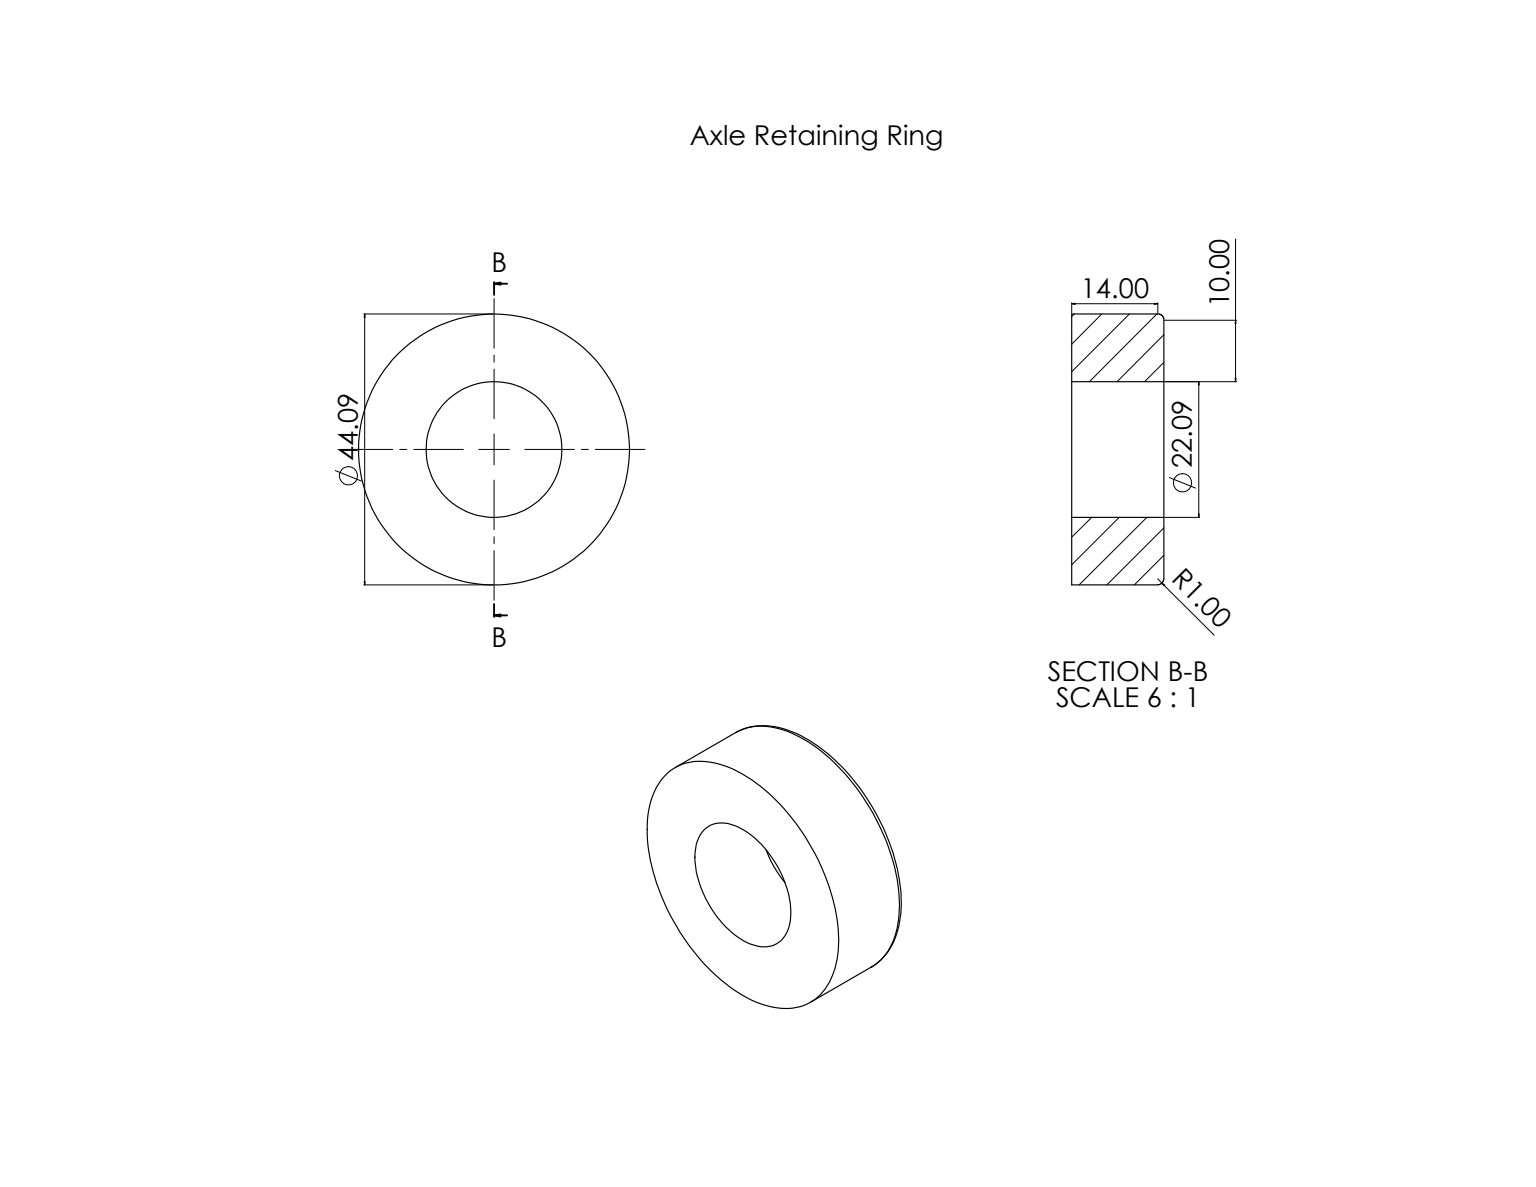
ISO-10303-21;
HEADER;
FILE_DESCRIPTION (('STEP AP214'),
    '1' );
FILE_NAME ('Axle Retaining Ring.step',
    '2026-10-21T18:33:49',
    ( '' ),
    ( '' ),
    'SwSTEP 2.0',
    'SolidWorks 2025',
    '' );
FILE_SCHEMA (( 'AUTOMOTIVE_DESIGN' ));
ENDSEC;

DATA;
#55=CIRCLE ( 'NONE', #2439, 22.04359719766050318 ) ;
#64=FACE_OUTER_BOUND ( 'NONE', #11864, .T. ) ;
#89=ORIENTED_EDGE ( 'NONE', *, *, #17144, .T. ) ;
#192=CYLINDRICAL_SURFACE ( 'NONE', #914, 11.04359719766050141 ) ;
#240=DIRECTION ( 'NONE',  ( 1.000000000000000000, 0.000000000000000000, 0.000000000000000000 ) ) ;
#257=MANIFOLD_SOLID_BREP ( 'Fillet4', #11497 ) ;
#347=SHAPE_REPRESENTATION_RELATIONSHIP ( 'NONE' , 'NONE' ,  #8623, #5245 ) ;
#437=ORIENTED_EDGE ( 'NONE', *, *, #1963, .T. ) ;
#454=DIRECTION ( 'NONE',  ( 0.000000000000000000, 0.000000000000000000, -1.000000000000000000 ) ) ;
#484=DIRECTION ( 'NONE',  ( 0.000000000000000000, 0.000000000000000000, -1.000000000000000000 ) ) ;
#549=FACE_OUTER_BOUND ( 'NONE', #11506, .T. ) ;
#746=DIRECTION ( 'NONE',  ( 0.000000000000000000, 0.000000000000000000, -1.000000000000000000 ) ) ;
#889=VERTEX_POINT ( 'NONE', #11533 ) ;
#914=AXIS2_PLACEMENT_3D ( 'NONE', #4475, #8427, #7036 ) ;
#1034=AXIS2_PLACEMENT_3D ( 'NONE', #3289, #4973, #4881 ) ;
#1044=DIRECTION ( 'NONE',  ( -1.000000000000000000, 0.000000000000000000, -0.000000000000000000 ) ) ;
#1046=STYLED_ITEM('',(#18559),#257);
#1223=CIRCLE ( 'NONE', #15253, 1.000000000000000888 ) ;
#1313=AXIS2_PLACEMENT_3D ( 'NONE', #12912, #7285, #17108 ) ;
#1444=EDGE_LOOP ( 'NONE', ( #12591, #14406, #8413, #6180 ) ) ;
#1515=DIRECTION ( 'NONE',  ( 1.000000000000000000, 0.000000000000000000, 0.000000000000000000 ) ) ;
#1526=VERTEX_POINT ( 'NONE', #2815 ) ;
#1551=DIRECTION ( 'NONE',  ( 0.000000000000000000, 0.000000000000000000, -1.000000000000000000 ) ) ;
#1578=DIRECTION ( 'NONE',  ( -1.224646799147353207E-16, 1.000000000000000000, 0.000000000000000000 ) ) ;
#1585=FACE_OUTER_BOUND ( 'NONE', #1876, .T. ) ;
#1605=FACE_OUTER_BOUND ( 'NONE', #1444, .T. ) ;
#1668=( NAMED_UNIT ( * ) PLANE_ANGLE_UNIT ( ) SI_UNIT ( $, .RADIAN. ) );
#1876=EDGE_LOOP ( 'NONE', ( #12983, #14667, #10558, #5358 ) ) ;
#1963=EDGE_CURVE ( 'NONE', #1526, #6914, #14518, .T. ) ;
#1995=EDGE_LOOP ( 'NONE', ( #11913, #4157 ) ) ;
#2070=AXIS2_PLACEMENT_3D ( 'NONE', #14552, #10073, #15773 ) ;
#2156=EDGE_CURVE ( 'NONE', #6914, #1526, #8158, .T. ) ;
#2191=VERTEX_POINT ( 'NONE', #5122 ) ;
#2398=DIRECTION ( 'NONE',  ( 0.000000000000000000, 0.000000000000000000, -1.000000000000000000 ) ) ;
#2439=AXIS2_PLACEMENT_3D ( 'NONE', #17290, #454, #8698 ) ;
#2806=AXIS2_PLACEMENT_3D ( 'NONE', #15914, #3105, #8818 ) ;
#2815=CARTESIAN_POINT ( 'NONE',  ( -46.03642545851250389, 84.22855780814606419, -47.50000000000000000 ) ) ;
#2834=CARTESIAN_POINT ( 'NONE',  ( -79.12361985383350316, 84.22855780814606419, -124.8487082408420861 ) ) ;
#2847=CARTESIAN_POINT ( 'NONE',  ( -57.08002265617300708, 84.22855780814606419, -61.50000000000000000 ) ) ;
#3105=DIRECTION ( 'NONE',  ( -0.000000000000000000, -0.000000000000000000, 1.000000000000000000 ) ) ;
#3289=CARTESIAN_POINT ( 'NONE',  ( -57.08002265617300708, 84.22855780814606419, -47.50000000000000000 ) ) ;
#3354=DIRECTION ( 'NONE',  ( 0.000000000000000000, 0.000000000000000000, -1.000000000000000000 ) ) ;
#3361=CARTESIAN_POINT ( 'NONE',  ( -68.12361985383350316, 84.22855780814606419, -124.8487082408420861 ) ) ;
#3368=DIRECTION ( 'NONE',  ( -1.000000000000000000, 0.000000000000000000, 0.000000000000000000 ) ) ;
#3372=AXIS2_PLACEMENT_3D ( 'NONE', #8660, #1551, #7259 ) ;
#3376=EDGE_CURVE ( 'NONE', #9602, #3839, #4404, .T. ) ;
#3486=ORIENTED_EDGE ( 'NONE', *, *, #18487, .F. ) ;
#3634=DIRECTION ( 'NONE',  ( -1.000000000000000000, 0.000000000000000000, 0.000000000000000000 ) ) ;
#3662=TOROIDAL_SURFACE ( 'NONE', #17400, 21.04359719766050674, 1.000000000000000000 ) ;
#3703=APPLICATION_CONTEXT ( 'automotive_design' ) ;
#3801=EDGE_CURVE ( 'NONE', #16706, #10794, #15822, .T. ) ;
#3839=VERTEX_POINT ( 'NONE', #7263 ) ;
#3840=PRODUCT_DEFINITION_CONTEXT ( 'detailed design', #3703, 'design' ) ;
#4157=ORIENTED_EDGE ( 'NONE', *, *, #3801, .T. ) ;
#4322=CYLINDRICAL_SURFACE ( 'NONE', #11999, 11.04359719766050141 ) ;
#4404=LINE ( 'NONE', #2834, #14606 ) ;
#4475=CARTESIAN_POINT ( 'NONE',  ( -57.08002265617300708, 84.22855780814606419, -124.8487082408420861 ) ) ;
#4610=CARTESIAN_POINT ( 'NONE',  ( -36.03642545851250389, 84.22855780814606419, -62.50000000000000000 ) ) ;
#4741=ADVANCED_FACE ( 'NONE', ( #5238, #6539 ), #16548, .T. ) ;
#4748=CARTESIAN_POINT ( 'NONE',  ( -57.08002265617300708, 84.22855780814606419, -47.50000000000000000 ) ) ;
#4881=DIRECTION ( 'NONE',  ( -1.000000000000000000, 0.000000000000000000, 0.000000000000000000 ) ) ;
#4901=ADVANCED_FACE ( 'NONE', ( #1585 ), #192, .F. ) ;
#4973=DIRECTION ( 'NONE',  ( 0.000000000000000000, 0.000000000000000000, -1.000000000000000000 ) ) ;
#5109=CARTESIAN_POINT ( 'NONE',  ( -78.12361985383350316, 84.22855780814606419, -61.50000000000000000 ) ) ;
#5122=CARTESIAN_POINT ( 'NONE',  ( -35.03642545851250389, 84.22855780814606419, -47.50000000000000000 ) ) ;
#5238=FACE_OUTER_BOUND ( 'NONE', #1995, .T. ) ;
#5245=ADVANCED_BREP_SHAPE_REPRESENTATION ( '', ( #257, #16217 ), #8171 ) ;
#5358=ORIENTED_EDGE ( 'NONE', *, *, #6020, .F. ) ;
#5466=CARTESIAN_POINT ( 'NONE',  ( -57.08002265617300708, 84.22855780814606419, -61.50000000000000000 ) ) ;
#5480=FACE_OUTER_BOUND ( 'NONE', #11849, .T. ) ;
#5519=AXIS2_PLACEMENT_3D ( 'NONE', #11491, #10346, #240 ) ;
#5637=ADVANCED_FACE ( 'NONE', ( #8637 ), #6191, .T. ) ;
#5675=EDGE_CURVE ( 'NONE', #3839, #2191, #17875, .T. ) ;
#5714=DIRECTION ( 'NONE',  ( -0.000000000000000000, -0.000000000000000000, 1.000000000000000000 ) ) ;
#5762=CYLINDRICAL_SURFACE ( 'NONE', #5519, 22.04359719766050318 ) ;
#5781=CARTESIAN_POINT ( 'NONE',  ( 0.000000000000000000, 0.000000000000000000, 0.000000000000000000 ) ) ;
#6020=EDGE_CURVE ( 'NONE', #9668, #1526, #13101, .T. ) ;
#6037=DIRECTION ( 'NONE',  ( 0.000000000000000000, 0.000000000000000000, 1.000000000000000000 ) ) ;
#6080=ORIENTED_EDGE ( 'NONE', *, *, #5675, .F. ) ;
#6180=ORIENTED_EDGE ( 'NONE', *, *, #2156, .F. ) ;
#6191=TOROIDAL_SURFACE ( 'NONE', #8622, 21.04359719766050674, 1.000000000000000000 ) ;
#6239=FACE_BOUND ( 'NONE', #11509, .T. ) ;
#6318=AXIS2_PLACEMENT_3D ( 'NONE', #5109, #15216, #2398 ) ;
#6347=VECTOR ( 'NONE', #13665, 1000.000000000000000 ) ;
#6352=CARTESIAN_POINT ( 'NONE',  ( -57.08002265617300708, 84.22855780814606419, -47.50000000000000000 ) ) ;
#6539=FACE_BOUND ( 'NONE', #11372, .T. ) ;
#6635=CARTESIAN_POINT ( 'NONE',  ( -46.03642545851250389, 84.22855780814606419, -62.50000000000000000 ) ) ;
#6740=CARTESIAN_POINT ( 'NONE',  ( -57.08002265617300708, 84.22855780814606419, -62.50000000000000000 ) ) ;
#6791=DIRECTION ( 'NONE',  ( -1.000000000000000000, 0.000000000000000000, -0.000000000000000000 ) ) ;
#6908=CIRCLE ( 'NONE', #12272, 22.04359719766050318 ) ;
#6914=VERTEX_POINT ( 'NONE', #16473 ) ;
#6923=CARTESIAN_POINT ( 'NONE',  ( -57.08002265617300708, 84.22855780814606419, -62.50000000000000000 ) ) ;
#7006=ORIENTED_EDGE ( 'NONE', *, *, #2156, .T. ) ;
#7012=DIRECTION ( 'NONE',  ( -0.000000000000000000, -0.000000000000000000, 1.000000000000000000 ) ) ;
#7036=DIRECTION ( 'NONE',  ( 1.000000000000000000, 0.000000000000000000, 0.000000000000000000 ) ) ;
#7099=LINE ( 'NONE', #18230, #12890 ) ;
#7259=DIRECTION ( 'NONE',  ( -1.000000000000000000, 0.000000000000000000, 0.000000000000000000 ) ) ;
#7263=CARTESIAN_POINT ( 'NONE',  ( -79.12361985383350316, 84.22855780814606419, -47.50000000000000000 ) ) ;
#7285=DIRECTION ( 'NONE',  ( 0.000000000000000000, 0.000000000000000000, -1.000000000000000000 ) ) ;
#7460=CARTESIAN_POINT ( 'NONE',  ( -57.08002265617300708, 84.22855780814606419, -61.50000000000000000 ) ) ;
#7481=PRODUCT_DEFINITION ( 'UNKNOWN', '', #9987, #3840 ) ;
#7550=( NAMED_UNIT ( * ) SI_UNIT ( $, .STERADIAN. ) SOLID_ANGLE_UNIT ( ) );
#7708=ORIENTED_EDGE ( 'NONE', *, *, #14542, .T. ) ;
#7914=CIRCLE ( 'NONE', #18390, 21.04359719766050318 ) ;
#7960=ORIENTED_EDGE ( 'NONE', *, *, #17144, .F. ) ;
#8036=DIRECTION ( 'NONE',  ( 0.000000000000000000, 0.000000000000000000, -1.000000000000000000 ) ) ;
#8158=CIRCLE ( 'NONE', #9073, 11.04359719766049430 ) ;
#8171=( GEOMETRIC_REPRESENTATION_CONTEXT ( 3 ) GLOBAL_UNCERTAINTY_ASSIGNED_CONTEXT ( ( #18256 ) ) GLOBAL_UNIT_ASSIGNED_CONTEXT ( ( #11672, #1668, #7550 ) ) REPRESENTATION_CONTEXT ( 'NONE', 'WORKASPACE' ) );
#8413=ORIENTED_EDGE ( 'NONE', *, *, #6020, .T. ) ;
#8425=CARTESIAN_POINT ( 'NONE',  ( -79.12361985383350316, 84.22855780814606419, -61.50000000000000000 ) ) ;
#8427=DIRECTION ( 'NONE',  ( -0.000000000000000000, -0.000000000000000000, 1.000000000000000000 ) ) ;
#8622=AXIS2_PLACEMENT_3D ( 'NONE', #2847, #15920, #17142 ) ;
#8623=SHAPE_REPRESENTATION ( 'Axle Retaining Ring', ( #16217 ), #8171 ) ;
#8630=ORIENTED_EDGE ( 'NONE', *, *, #12433, .F. ) ;
#8637=FACE_OUTER_BOUND ( 'NONE', #14875, .T. ) ;
#8660=CARTESIAN_POINT ( 'NONE',  ( -57.08002265617300708, 84.22855780814606419, -62.50000000000000000 ) ) ;
#8698=DIRECTION ( 'NONE',  ( -1.000000000000000000, 0.000000000000000000, 0.000000000000000000 ) ) ;
#8803=MECHANICAL_DESIGN_GEOMETRIC_PRESENTATION_REPRESENTATION('',(#1046),#17447);
#8818=DIRECTION ( 'NONE',  ( -1.000000000000000000, 0.000000000000000000, 0.000000000000000000 ) ) ;
#8961=DIRECTION ( 'NONE',  ( 1.000000000000000000, 0.000000000000000000, 0.000000000000000000 ) ) ;
#9073=AXIS2_PLACEMENT_3D ( 'NONE', #13654, #746, #17658 ) ;
#9365=ADVANCED_FACE ( 'NONE', ( #1605 ), #4322, .F. ) ;
#9441=APPLICATION_CONTEXT ( 'automotive_design' ) ;
#9448=DIRECTION ( 'NONE',  ( 0.000000000000000000, 0.000000000000000000, -1.000000000000000000 ) ) ;
#9602=VERTEX_POINT ( 'NONE', #8425 ) ;
#9668=VERTEX_POINT ( 'NONE', #6635 ) ;
#9956=( LENGTH_UNIT ( ) NAMED_UNIT ( * ) SI_UNIT ( .MILLI., .METRE. ) );
#9987=PRODUCT_DEFINITION_FORMATION_WITH_SPECIFIED_SOURCE ( 'ANY', '', #17885, .NOT_KNOWN. ) ;
#10046=ORIENTED_EDGE ( 'NONE', *, *, #17180, .T. ) ;
#10073=DIRECTION ( 'NONE',  ( 0.000000000000000000, 0.000000000000000000, -1.000000000000000000 ) ) ;
#10084=ADVANCED_FACE ( 'NONE', ( #18196 ), #3662, .T. ) ;
#10346=DIRECTION ( 'NONE',  ( -0.000000000000000000, -0.000000000000000000, 1.000000000000000000 ) ) ;
#10467=AXIS2_PLACEMENT_3D ( 'NONE', #6740, #8036, #1044 ) ;
#10558=ORIENTED_EDGE ( 'NONE', *, *, #1963, .F. ) ;
#10630=EDGE_CURVE ( 'NONE', #9602, #11331, #14443, .T. ) ;
#10651=EDGE_CURVE ( 'NONE', #889, #6914, #15055, .T. ) ;
#10728=ORIENTED_EDGE ( 'NONE', *, *, #3376, .F. ) ;
#10794=VERTEX_POINT ( 'NONE', #15015 ) ;
#11011=ADVANCED_FACE ( 'NONE', ( #5480 ), #11207, .T. ) ;
#11114=EDGE_CURVE ( 'NONE', #9668, #889, #16838, .T. ) ;
#11207=CYLINDRICAL_SURFACE ( 'NONE', #18036, 22.04359719766050318 ) ;
#11323=ORIENTED_EDGE ( 'NONE', *, *, #15890, .T. ) ;
#11331=VERTEX_POINT ( 'NONE', #11592 ) ;
#11372=EDGE_LOOP ( 'NONE', ( #14308, #3486 ) ) ;
#11428=DIRECTION ( 'NONE',  ( -0.000000000000000000, -0.000000000000000000, 1.000000000000000000 ) ) ;
#11491=CARTESIAN_POINT ( 'NONE',  ( -57.08002265617300708, 84.22855780814606419, -124.8487082408420861 ) ) ;
#11497=CLOSED_SHELL ( 'NONE', ( #5637, #4901, #11011, #11787, #12967, #9365, #4741, #10084 ) ) ;
#11506=EDGE_LOOP ( 'NONE', ( #7960, #6080 ) ) ;
#11509=EDGE_LOOP ( 'NONE', ( #437, #7006 ) ) ;
#11533=CARTESIAN_POINT ( 'NONE',  ( -68.12361985383350316, 84.22855780814606419, -62.50000000000000000 ) ) ;
#11592=CARTESIAN_POINT ( 'NONE',  ( -35.03642545851250389, 84.22855780814606419, -61.50000000000000000 ) ) ;
#11672=( LENGTH_UNIT ( ) NAMED_UNIT ( * ) SI_UNIT ( .MILLI., .METRE. ) );
#11678=CARTESIAN_POINT ( 'NONE',  ( -36.03642545851250389, 84.22855780814606419, -61.50000000000000000 ) ) ;
#11787=ADVANCED_FACE ( 'NONE', ( #64 ), #5762, .T. ) ;
#11849=EDGE_LOOP ( 'NONE', ( #12289, #18252, #13254, #12189 ) ) ;
#11864=EDGE_LOOP ( 'NONE', ( #10728, #13849, #7708, #89 ) ) ;
#11913=ORIENTED_EDGE ( 'NONE', *, *, #12433, .T. ) ;
#11999=AXIS2_PLACEMENT_3D ( 'NONE', #15820, #5714, #1515 ) ;
#12076=ORIENTED_EDGE ( 'NONE', *, *, #15923, .F. ) ;
#12189=ORIENTED_EDGE ( 'NONE', *, *, #14542, .F. ) ;
#12272=AXIS2_PLACEMENT_3D ( 'NONE', #7460, #17283, #14660 ) ;
#12289=ORIENTED_EDGE ( 'NONE', *, *, #15923, .T. ) ;
#12317=CIRCLE ( 'NONE', #6318, 1.000000000000000888 ) ;
#12405=SHAPE_DEFINITION_REPRESENTATION ( #12710, #8623 ) ;
#12433=EDGE_CURVE ( 'NONE', #10794, #16706, #7914, .T. ) ;
#12591=ORIENTED_EDGE ( 'NONE', *, *, #10651, .F. ) ;
#12710=PRODUCT_DEFINITION_SHAPE ( 'NONE', 'NONE',  #7481 ) ;
#12890=VECTOR ( 'NONE', #7012, 1000.000000000000000 ) ;
#12912=CARTESIAN_POINT ( 'NONE',  ( -57.08002265617300708, 84.22855780814606419, -62.50000000000000000 ) ) ;
#12967=ADVANCED_FACE ( 'NONE', ( #549, #6239 ), #17566, .F. ) ;
#12983=ORIENTED_EDGE ( 'NONE', *, *, #11114, .T. ) ;
#13070=DIRECTION ( 'NONE',  ( 1.000000000000000000, 0.000000000000000000, 0.000000000000000000 ) ) ;
#13101=LINE ( 'NONE', #14322, #15796 ) ;
#13254=ORIENTED_EDGE ( 'NONE', *, *, #5675, .T. ) ;
#13299=ORIENTED_EDGE ( 'NONE', *, *, #3801, .F. ) ;
#13391=UNCERTAINTY_MEASURE_WITH_UNIT (LENGTH_MEASURE( 1.000000000000000082E-05 ), #9956, 'distance_accuracy_value', 'NONE');
#13654=CARTESIAN_POINT ( 'NONE',  ( -57.08002265617300708, 84.22855780814606419, -47.50000000000000000 ) ) ;
#13665=DIRECTION ( 'NONE',  ( -0.000000000000000000, -0.000000000000000000, 1.000000000000000000 ) ) ;
#13849=ORIENTED_EDGE ( 'NONE', *, *, #10630, .T. ) ;
#13996=DIRECTION ( 'NONE',  ( -1.000000000000000000, 0.000000000000000000, 0.000000000000000000 ) ) ;
#14308=ORIENTED_EDGE ( 'NONE', *, *, #11114, .F. ) ;
#14322=CARTESIAN_POINT ( 'NONE',  ( -46.03642545851250389, 84.22855780814606419, -124.8487082408420861 ) ) ;
#14406=ORIENTED_EDGE ( 'NONE', *, *, #18487, .T. ) ;
#14443=CIRCLE ( 'NONE', #2806, 22.04359719766050318 ) ;
#14518=CIRCLE ( 'NONE', #1034, 11.04359719766049430 ) ;
#14542=EDGE_CURVE ( 'NONE', #11331, #2191, #7099, .T. ) ;
#14552=CARTESIAN_POINT ( 'NONE',  ( -57.08002265617300708, 84.22855780814606419, -62.50000000000000000 ) ) ;
#14606=VECTOR ( 'NONE', #17301, 1000.000000000000000 ) ;
#14660=DIRECTION ( 'NONE',  ( -1.000000000000000000, 0.000000000000000000, 0.000000000000000000 ) ) ;
#14667=ORIENTED_EDGE ( 'NONE', *, *, #10651, .T. ) ;
#14875=EDGE_LOOP ( 'NONE', ( #12076, #11323, #8630, #16662 ) ) ;
#15015=CARTESIAN_POINT ( 'NONE',  ( -78.12361985383350316, 84.22855780814606419, -62.50000000000000000 ) ) ;
#15055=LINE ( 'NONE', #3361, #6347 ) ;
#15179=PRODUCT_CONTEXT ( 'NONE', #9441, 'mechanical' ) ;
#15216=DIRECTION ( 'NONE',  ( -0.000000000000000000, -1.000000000000000000, -0.000000000000000000 ) ) ;
#15253=AXIS2_PLACEMENT_3D ( 'NONE', #11678, #1578, #17466 ) ;
#15273=ORIENTED_EDGE ( 'NONE', *, *, #15890, .F. ) ;
#15277=( NAMED_UNIT ( * ) PLANE_ANGLE_UNIT ( ) SI_UNIT ( $, .RADIAN. ) );
#15418=AXIS2_PLACEMENT_3D ( 'NONE', #4748, #3354, #6791 ) ;
#15473=( NAMED_UNIT ( * ) SI_UNIT ( $, .STERADIAN. ) SOLID_ANGLE_UNIT ( ) );
#15773=DIRECTION ( 'NONE',  ( -1.000000000000000000, 0.000000000000000000, 0.000000000000000000 ) ) ;
#15796=VECTOR ( 'NONE', #11428, 1000.000000000000000 ) ;
#15820=CARTESIAN_POINT ( 'NONE',  ( -57.08002265617300708, 84.22855780814606419, -124.8487082408420861 ) ) ;
#15822=CIRCLE ( 'NONE', #2070, 21.04359719766050318 ) ;
#15890=EDGE_CURVE ( 'NONE', #11331, #16706, #1223, .T. ) ;
#15914=CARTESIAN_POINT ( 'NONE',  ( -57.08002265617300708, 84.22855780814606419, -61.50000000000000000 ) ) ;
#15920=DIRECTION ( 'NONE',  ( 0.000000000000000000, 0.000000000000000000, -1.000000000000000000 ) ) ;
#15923=EDGE_CURVE ( 'NONE', #11331, #9602, #6908, .T. ) ;
#16217=AXIS2_PLACEMENT_3D ( 'NONE', #5781, #6037, #8961 ) ;
#16473=CARTESIAN_POINT ( 'NONE',  ( -68.12361985383350316, 84.22855780814606419, -47.50000000000000000 ) ) ;
#16548=PLANE ( 'NONE',  #10467 ) ;
#16662=ORIENTED_EDGE ( 'NONE', *, *, #17180, .F. ) ;
#16706=VERTEX_POINT ( 'NONE', #4610 ) ;
#16776=DIRECTION ( 'NONE',  ( 0.000000000000000000, 0.000000000000000000, -1.000000000000000000 ) ) ;
#16838=CIRCLE ( 'NONE', #3372, 11.04359719766049430 ) ;
#17108=DIRECTION ( 'NONE',  ( -1.000000000000000000, 0.000000000000000000, 0.000000000000000000 ) ) ;
#17142=DIRECTION ( 'NONE',  ( -1.000000000000000000, 0.000000000000000000, 0.000000000000000000 ) ) ;
#17144=EDGE_CURVE ( 'NONE', #2191, #3839, #55, .T. ) ;
#17148=EDGE_LOOP ( 'NONE', ( #15273, #18466, #10046, #13299 ) ) ;
#17180=EDGE_CURVE ( 'NONE', #9602, #10794, #12317, .T. ) ;
#17253=DIRECTION ( 'NONE',  ( -0.000000000000000000, -0.000000000000000000, 1.000000000000000000 ) ) ;
#17283=DIRECTION ( 'NONE',  ( -0.000000000000000000, -0.000000000000000000, 1.000000000000000000 ) ) ;
#17290=CARTESIAN_POINT ( 'NONE',  ( -57.08002265617300708, 84.22855780814606419, -47.50000000000000000 ) ) ;
#17301=DIRECTION ( 'NONE',  ( -0.000000000000000000, -0.000000000000000000, 1.000000000000000000 ) ) ;
#17400=AXIS2_PLACEMENT_3D ( 'NONE', #5466, #16776, #13996 ) ;
#17408=CIRCLE ( 'NONE', #1313, 11.04359719766049430 ) ;
#17433=CARTESIAN_POINT ( 'NONE',  ( -57.08002265617300708, 84.22855780814606419, -124.8487082408420861 ) ) ;
#17447=( GEOMETRIC_REPRESENTATION_CONTEXT ( 3 ) GLOBAL_UNCERTAINTY_ASSIGNED_CONTEXT ( ( #13391 ) ) GLOBAL_UNIT_ASSIGNED_CONTEXT ( ( #9956, #15277, #15473 ) ) REPRESENTATION_CONTEXT ( 'NONE', 'WORKASPACE' ) );
#17466=DIRECTION ( 'NONE',  ( -1.000000000000000000, 0.000000000000000000, 0.000000000000000000 ) ) ;
#17566=PLANE ( 'NONE',  #15418 ) ;
#17658=DIRECTION ( 'NONE',  ( -1.000000000000000000, 0.000000000000000000, 0.000000000000000000 ) ) ;
#17875=CIRCLE ( 'NONE', #18184, 22.04359719766050318 ) ;
#17885=PRODUCT ( 'Axle Retaining Ring', 'Axle Retaining Ring', '', ( #15179 ) ) ;
#18036=AXIS2_PLACEMENT_3D ( 'NONE', #17433, #17253, #13070 ) ;
#18184=AXIS2_PLACEMENT_3D ( 'NONE', #6352, #484, #3368 ) ;
#18196=FACE_OUTER_BOUND ( 'NONE', #17148, .T. ) ;
#18230=CARTESIAN_POINT ( 'NONE',  ( -35.03642545851250389, 84.22855780814606419, -124.8487082408420861 ) ) ;
#18252=ORIENTED_EDGE ( 'NONE', *, *, #3376, .T. ) ;
#18256=UNCERTAINTY_MEASURE_WITH_UNIT (LENGTH_MEASURE( 1.000000000000000082E-05 ), #11672, 'distance_accuracy_value', 'NONE');
#18390=AXIS2_PLACEMENT_3D ( 'NONE', #6923, #9448, #3634 ) ;
#18466=ORIENTED_EDGE ( 'NONE', *, *, #10630, .F. ) ;
#18487=EDGE_CURVE ( 'NONE', #889, #9668, #17408, .T. ) ;
#18553=COLOUR_RGB('Grey',0.48,0.52,0.57);
#18554=FILL_AREA_STYLE_COLOUR('',#18553);
#18555=FILL_AREA_STYLE('',(#18554));
#18556=SURFACE_STYLE_FILL_AREA(#18555);
#18557=SURFACE_SIDE_STYLE('',(#18556));
#18558=SURFACE_STYLE_USAGE(.BOTH.,#18557);
#18559=PRESENTATION_STYLE_ASSIGNMENT((#18558));
ENDSEC;
END-ISO-10303-21;
